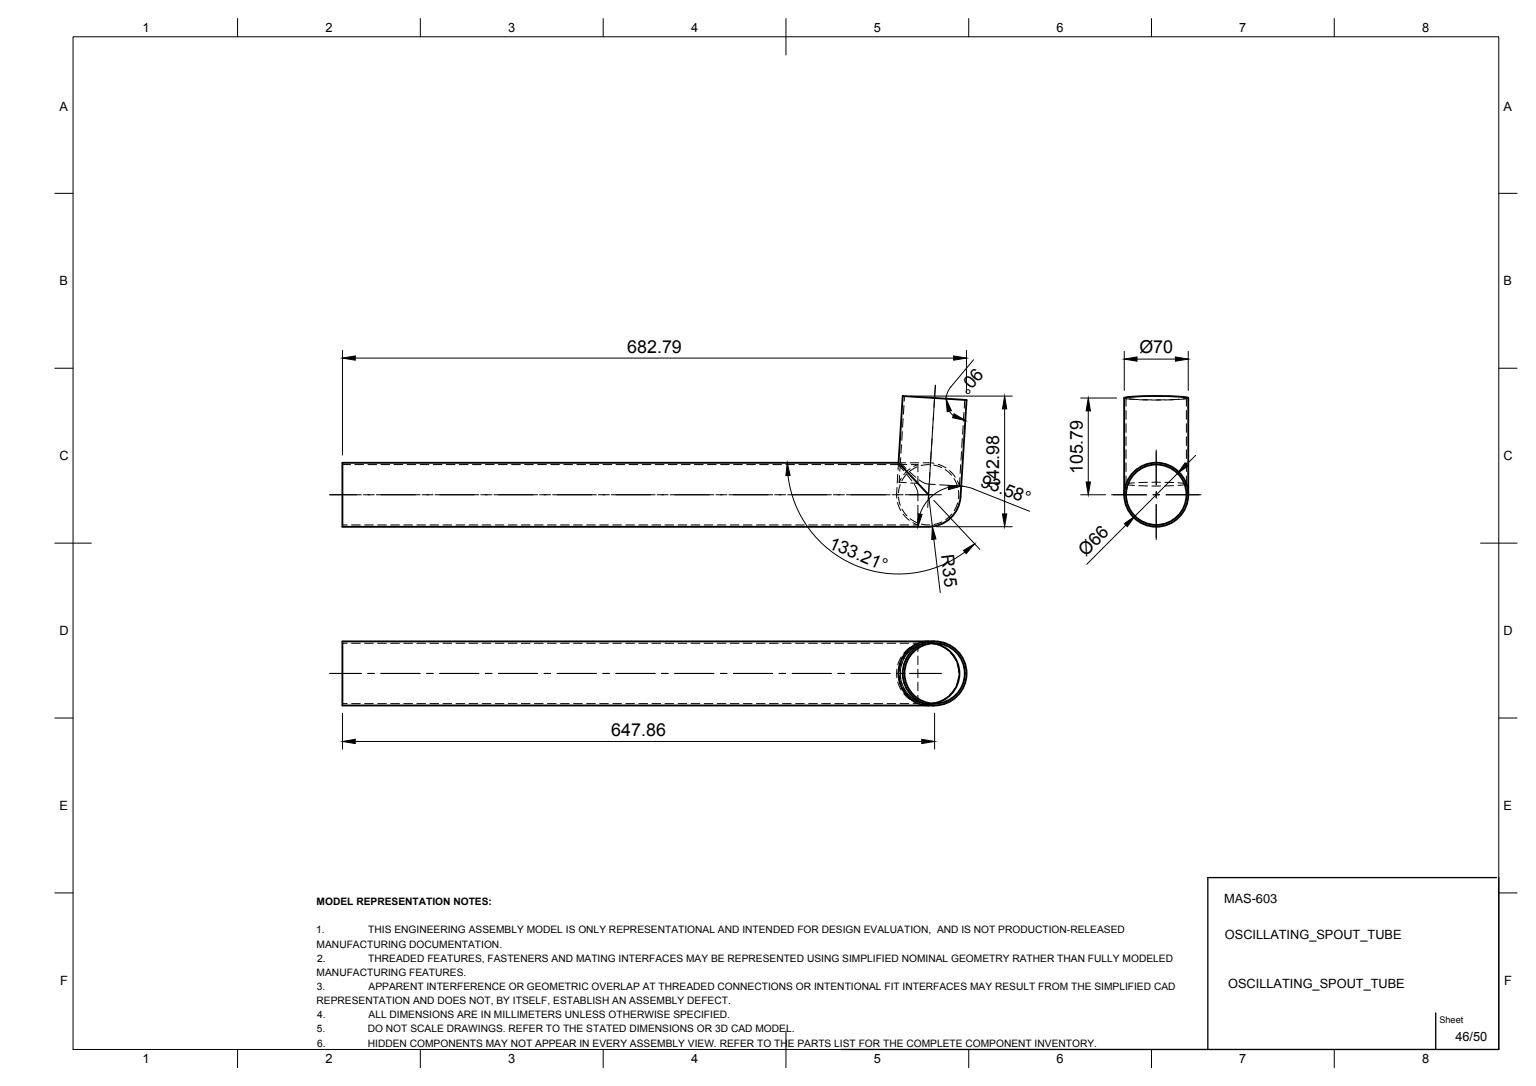
ISO-10303-21;
HEADER;
FILE_DESCRIPTION((''),'2;1');
FILE_NAME('OSCILLATING_SPOUT_TUBE.step','2026-10-01T22:06:14-07:00',(''),(''),'','','');
FILE_SCHEMA (('AUTOMOTIVE_DESIGN { 1 0 10303 214 3 1 1 }'));
ENDSEC;
DATA;
#10=MECHANICAL_DESIGN_GEOMETRIC_PRESENTATION_REPRESENTATION('',(#1021),#50440);
#36=B_SPLINE_CURVE_WITH_KNOTS('',3,(#49390,#49391,#49392,#49393,#49394,
#49395,#49396,#49397,#49398,#49399,#49400,#49401,#49402,#49403,#49404,#49405,
#49406,#49407,#49408,#49409,#49410,#49411,#49412,#49413,#49414,#49415,#49416,
#49417,#49418,#49419,#49420,#49421,#49422,#49423,#49424,#49425,#49426,#49427),
 .UNSPECIFIED.,.F.,.F.,(4,2,2,2,2,2,2,2,2,2,2,2,2,2,2,2,2,2,4),(11.701609895415,
11.9954810277209,12.363235333761,13.0987439458412,13.8342525579214,14.5697611700016,
15.2442090288987,15.9186568877959,16.593104746693,17.2675526055902,17.9420004644874,
18.6164483233845,19.2908961822817,19.9653440411788,20.700852653259,21.4363612653392,
22.1718698774194,22.5396241834595,22.8334953157654),.UNSPECIFIED.) ;
#37=B_SPLINE_CURVE_WITH_KNOTS('',3,(#49445,#49446,#49447,#49448,#49449,
#49450,#49451,#49452,#49453,#49454,#49455,#49456,#49457,#49458,#49459,#49460,
#49461,#49462,#49463,#49464,#49465,#49466,#49467,#49468,#49469,#49470,#49471,
#49472,#49473,#49474,#49475,#49476,#49477,#49478,#49479,#49480,#49481,#49482),
 .UNSPECIFIED.,.F.,.F.,(4,2,2,2,2,2,2,2,2,2,2,2,2,2,2,2,2,2,4),(0.0738831737341421,
0.367754306040092,0.735508612080185,1.47101722416037,2.20652583624055,2.94203444832074,
3.61648230721789,4.29093016611505,4.9653780250122,5.63982588390936,6.31427374280651,
6.98872160170367,7.66316946060082,8.33761731949797,9.07312593157816,9.80863454365834,
10.5441431557385,10.9118974617786,11.2057685940846),.UNSPECIFIED.) ;
#77=ORIENTED_CLOSED_SHELL('',*,#28697,.F.) ;
#78=ORIENTED_CLOSED_SHELL('',*,#28698,.F.) ;
#81=BREP_WITH_VOIDS('OSCILLATING_SPOUT_TUBE',#28699,(#77,#78)) ;
#673=ELLIPSE('',#32089,4.52782199571862,3.3) ;
#674=ELLIPSE('',#32097,4.80223545000459,3.5) ;
#875=SPHERICAL_SURFACE('',#32083,3.3) ;
#876=SPHERICAL_SURFACE('',#32085,3.5) ;
#877=SPHERICAL_SURFACE('',#32114,3.5) ;
#878=SPHERICAL_SURFACE('',#32115,3.5) ;
#879=SPHERICAL_SURFACE('',#32116,3.5) ;
#924=SHAPE_REPRESENTATION_RELATIONSHIP('SRR','None',#50658,#969) ;
#969=ADVANCED_BREP_SHAPE_REPRESENTATION('',(#81),#50427) ;
#1021=STYLED_ITEM('',(#50889),#81) ;
#1388=FACE_BOUND('',#5587,.T.) ;
#1389=FACE_BOUND('',#5591,.T.) ;
#2256=PLANE('',#32091) ;
#2257=PLANE('',#32100) ;
#3752=FACE_OUTER_BOUND('',#5582,.T.) ;
#3753=FACE_OUTER_BOUND('',#5583,.T.) ;
#3754=FACE_OUTER_BOUND('',#5584,.T.) ;
#3755=FACE_OUTER_BOUND('',#5585,.T.) ;
#3756=FACE_OUTER_BOUND('',#5586,.T.) ;
#3757=FACE_OUTER_BOUND('',#5588,.T.) ;
#3758=FACE_OUTER_BOUND('',#5589,.T.) ;
#3759=FACE_OUTER_BOUND('',#5590,.T.) ;
#3760=FACE_OUTER_BOUND('',#5592,.T.) ;
#3761=FACE_OUTER_BOUND('',#5593,.T.) ;
#3762=FACE_OUTER_BOUND('',#5594,.T.) ;
#3763=FACE_OUTER_BOUND('',#5595,.T.) ;
#3764=FACE_OUTER_BOUND('',#5596,.T.) ;
#3765=FACE_OUTER_BOUND('',#5597,.T.) ;
#3766=FACE_OUTER_BOUND('',#5598,.T.) ;
#5582=EDGE_LOOP('',(#26027,#26028)) ;
#5583=EDGE_LOOP('',(#26029,#26030)) ;
#5584=EDGE_LOOP('',(#26031,#26032)) ;
#5585=EDGE_LOOP('',(#26033,#26034)) ;
#5586=EDGE_LOOP('',(#26035)) ;
#5587=EDGE_LOOP('',(#26036)) ;
#5588=EDGE_LOOP('',(#26037,#26038)) ;
#5589=EDGE_LOOP('',(#26039,#26040,#26041,#26042,#26043,#26044)) ;
#5590=EDGE_LOOP('',(#26045)) ;
#5591=EDGE_LOOP('',(#26046)) ;
#5592=EDGE_LOOP('',(#26047,#26048)) ;
#5593=EDGE_LOOP('',(#26049,#26050,#26051,#26052,#26053,#26054)) ;
#5594=EDGE_LOOP('',(#26055,#26056,#26057,#26058,#26059,#26060)) ;
#5595=EDGE_LOOP('',(#26061,#26062,#26063,#26064,#26065,#26066)) ;
#5596=EDGE_LOOP('',(#26067,#26068,#26069)) ;
#5597=EDGE_LOOP('',(#26070,#26071,#26072,#26073)) ;
#5598=EDGE_LOOP('',(#26074,#26075,#26076,#26077,#26078)) ;
#8039=LINE('',#49435,#10511) ;
#8040=LINE('',#49486,#10512) ;
#8041=LINE('',#49492,#10513) ;
#8042=LINE('',#49496,#10514) ;
#10511=VECTOR('',#40462,3.5) ;
#10512=VECTOR('',#40477,3.5) ;
#10513=VECTOR('',#40486,3.3) ;
#10514=VECTOR('',#40491,3.3) ;
#11759=CIRCLE('',#32084,3.3) ;
#11760=CIRCLE('',#32086,3.3) ;
#11761=CIRCLE('',#32087,3.3) ;
#11762=CIRCLE('',#32092,3.5) ;
#11763=CIRCLE('',#32093,3.3) ;
#11764=CIRCLE('',#32095,3.5) ;
#11765=CIRCLE('',#32098,3.5) ;
#11766=CIRCLE('',#32099,3.5) ;
#11767=CIRCLE('',#32101,3.5) ;
#11768=CIRCLE('',#32102,3.3) ;
#11769=CIRCLE('',#32104,3.5) ;
#11770=CIRCLE('',#32106,3.5) ;
#11771=CIRCLE('',#32107,3.5) ;
#11772=CIRCLE('',#32109,3.3) ;
#11773=CIRCLE('',#32110,3.3) ;
#11774=CIRCLE('',#32112,3.3) ;
#11775=CIRCLE('',#32113,3.3) ;
#11776=CIRCLE('',#32117,3.5) ;
#14351=VERTEX_POINT('',#49371) ;
#14352=VERTEX_POINT('',#49372) ;
#14353=VERTEX_POINT('',#49375) ;
#14354=VERTEX_POINT('',#49376) ;
#14355=VERTEX_POINT('',#49383) ;
#14356=VERTEX_POINT('',#49385) ;
#14357=VERTEX_POINT('',#49388) ;
#14358=VERTEX_POINT('',#49389) ;
#14359=VERTEX_POINT('',#49430) ;
#14360=VERTEX_POINT('',#49431) ;
#14361=VERTEX_POINT('',#49433) ;
#14362=VERTEX_POINT('',#49438) ;
#14363=VERTEX_POINT('',#49440) ;
#14364=VERTEX_POINT('',#49443) ;
#14365=VERTEX_POINT('',#49444) ;
#14366=VERTEX_POINT('',#49485) ;
#14367=VERTEX_POINT('',#49490) ;
#14368=VERTEX_POINT('',#49495) ;
#14369=VERTEX_POINT('',#49502) ;
#18279=EDGE_CURVE('',#14351,#14352,#11759,.T.) ;
#18280=EDGE_CURVE('',#14353,#14354,#11760,.T.) ;
#18281=EDGE_CURVE('',#14354,#14353,#11761,.T.) ;
#18282=EDGE_CURVE('',#14353,#14354,#673,.T.) ;
#18283=EDGE_CURVE('',#14355,#14355,#11762,.T.) ;
#18284=EDGE_CURVE('',#14356,#14356,#11763,.T.) ;
#18285=EDGE_CURVE('',#14357,#14358,#36,.T.) ;
#18286=EDGE_CURVE('',#14357,#14358,#11764,.T.) ;
#18287=EDGE_CURVE('',#14359,#14360,#674,.T.) ;
#18288=EDGE_CURVE('',#14361,#14360,#11765,.T.) ;
#18289=EDGE_CURVE('',#14361,#14355,#8039,.T.) ;
#18290=EDGE_CURVE('',#14359,#14361,#11766,.T.) ;
#18291=EDGE_CURVE('',#14362,#14362,#11767,.T.) ;
#18292=EDGE_CURVE('',#14363,#14363,#11768,.T.) ;
#18293=EDGE_CURVE('',#14364,#14365,#37,.T.) ;
#18294=EDGE_CURVE('',#14365,#14364,#11769,.T.) ;
#18295=EDGE_CURVE('',#14362,#14366,#8040,.T.) ;
#18296=EDGE_CURVE('',#14360,#14366,#11770,.T.) ;
#18297=EDGE_CURVE('',#14366,#14359,#11771,.T.) ;
#18298=EDGE_CURVE('',#14357,#14367,#11772,.T.) ;
#18299=EDGE_CURVE('',#14367,#14363,#8041,.T.) ;
#18300=EDGE_CURVE('',#14367,#14358,#11773,.T.) ;
#18301=EDGE_CURVE('',#14356,#14368,#8042,.T.) ;
#18302=EDGE_CURVE('',#14368,#14364,#11774,.T.) ;
#18303=EDGE_CURVE('',#14365,#14368,#11775,.T.) ;
#18304=EDGE_CURVE('',#14369,#14368,#11776,.T.) ;
#26027=ORIENTED_EDGE('',*,*,#18279,.T.) ;
#26028=ORIENTED_EDGE('',*,*,#18279,.F.) ;
#26029=ORIENTED_EDGE('',*,*,#18280,.F.) ;
#26030=ORIENTED_EDGE('',*,*,#18281,.F.) ;
#26031=ORIENTED_EDGE('',*,*,#18281,.T.) ;
#26032=ORIENTED_EDGE('',*,*,#18282,.T.) ;
#26033=ORIENTED_EDGE('',*,*,#18280,.T.) ;
#26034=ORIENTED_EDGE('',*,*,#18282,.F.) ;
#26035=ORIENTED_EDGE('',*,*,#18283,.T.) ;
#26036=ORIENTED_EDGE('',*,*,#18284,.T.) ;
#26037=ORIENTED_EDGE('',*,*,#18285,.T.) ;
#26038=ORIENTED_EDGE('',*,*,#18286,.F.) ;
#26039=ORIENTED_EDGE('',*,*,#18287,.T.) ;
#26040=ORIENTED_EDGE('',*,*,#18288,.F.) ;
#26041=ORIENTED_EDGE('',*,*,#18289,.T.) ;
#26042=ORIENTED_EDGE('',*,*,#18283,.F.) ;
#26043=ORIENTED_EDGE('',*,*,#18289,.F.) ;
#26044=ORIENTED_EDGE('',*,*,#18290,.F.) ;
#26045=ORIENTED_EDGE('',*,*,#18291,.T.) ;
#26046=ORIENTED_EDGE('',*,*,#18292,.T.) ;
#26047=ORIENTED_EDGE('',*,*,#18293,.F.) ;
#26048=ORIENTED_EDGE('',*,*,#18294,.F.) ;
#26049=ORIENTED_EDGE('',*,*,#18291,.F.) ;
#26050=ORIENTED_EDGE('',*,*,#18295,.T.) ;
#26051=ORIENTED_EDGE('',*,*,#18296,.F.) ;
#26052=ORIENTED_EDGE('',*,*,#18287,.F.) ;
#26053=ORIENTED_EDGE('',*,*,#18297,.F.) ;
#26054=ORIENTED_EDGE('',*,*,#18295,.F.) ;
#26055=ORIENTED_EDGE('',*,*,#18298,.T.) ;
#26056=ORIENTED_EDGE('',*,*,#18299,.T.) ;
#26057=ORIENTED_EDGE('',*,*,#18292,.F.) ;
#26058=ORIENTED_EDGE('',*,*,#18299,.F.) ;
#26059=ORIENTED_EDGE('',*,*,#18300,.T.) ;
#26060=ORIENTED_EDGE('',*,*,#18285,.F.) ;
#26061=ORIENTED_EDGE('',*,*,#18284,.F.) ;
#26062=ORIENTED_EDGE('',*,*,#18301,.T.) ;
#26063=ORIENTED_EDGE('',*,*,#18302,.T.) ;
#26064=ORIENTED_EDGE('',*,*,#18293,.T.) ;
#26065=ORIENTED_EDGE('',*,*,#18303,.T.) ;
#26066=ORIENTED_EDGE('',*,*,#18301,.F.) ;
#26067=ORIENTED_EDGE('',*,*,#18298,.F.) ;
#26068=ORIENTED_EDGE('',*,*,#18286,.T.) ;
#26069=ORIENTED_EDGE('',*,*,#18300,.F.) ;
#26070=ORIENTED_EDGE('',*,*,#18296,.T.) ;
#26071=ORIENTED_EDGE('',*,*,#18297,.T.) ;
#26072=ORIENTED_EDGE('',*,*,#18290,.T.) ;
#26073=ORIENTED_EDGE('',*,*,#18288,.T.) ;
#26074=ORIENTED_EDGE('',*,*,#18294,.T.) ;
#26075=ORIENTED_EDGE('',*,*,#18302,.F.) ;
#26076=ORIENTED_EDGE('',*,*,#18304,.F.) ;
#26077=ORIENTED_EDGE('',*,*,#18304,.T.) ;
#26078=ORIENTED_EDGE('',*,*,#18303,.F.) ;
#27033=CYLINDRICAL_SURFACE('',#32088,3.3) ;
#27034=CYLINDRICAL_SURFACE('',#32090,3.3) ;
#27035=CYLINDRICAL_SURFACE('',#32094,3.5) ;
#27036=CYLINDRICAL_SURFACE('',#32096,3.5) ;
#27037=CYLINDRICAL_SURFACE('',#32103,3.5) ;
#27038=CYLINDRICAL_SURFACE('',#32105,3.5) ;
#27039=CYLINDRICAL_SURFACE('',#32108,3.3) ;
#27040=CYLINDRICAL_SURFACE('',#32111,3.3) ;
#28487=ADVANCED_FACE('',(#3752),#875,.F.) ;
#28488=ADVANCED_FACE('',(#3753),#876,.T.) ;
#28489=ADVANCED_FACE('',(#3754),#27033,.F.) ;
#28490=ADVANCED_FACE('',(#3755),#27034,.F.) ;
#28491=ADVANCED_FACE('',(#3756,#1388),#2256,.T.) ;
#28492=ADVANCED_FACE('',(#3757),#27035,.T.) ;
#28493=ADVANCED_FACE('',(#3758),#27036,.T.) ;
#28494=ADVANCED_FACE('',(#3759,#1389),#2257,.T.) ;
#28495=ADVANCED_FACE('',(#3760),#27037,.T.) ;
#28496=ADVANCED_FACE('',(#3761),#27038,.T.) ;
#28497=ADVANCED_FACE('',(#3762),#27039,.F.) ;
#28498=ADVANCED_FACE('',(#3763),#27040,.F.) ;
#28499=ADVANCED_FACE('',(#3764),#877,.T.) ;
#28500=ADVANCED_FACE('',(#3765),#878,.T.) ;
#28501=ADVANCED_FACE('',(#3766),#879,.T.) ;
#28697=CLOSED_SHELL('',(#28487)) ;
#28698=CLOSED_SHELL('',(#28488,#28489,#28490)) ;
#28699=CLOSED_SHELL('',(#28491,#28492,#28493,#28494,#28495,#28496,#28497,
#28498,#28499,#28500,#28501)) ;
#32082=AXIS2_PLACEMENT_3D('',#49369,#40428,#40429) ;
#32083=AXIS2_PLACEMENT_3D('',#49370,#40430,#40431) ;
#32084=AXIS2_PLACEMENT_3D('',#49373,#40432,#40433) ;
#32085=AXIS2_PLACEMENT_3D('',#49374,#40434,#40435) ;
#32086=AXIS2_PLACEMENT_3D('',#49377,#40436,#40437) ;
#32087=AXIS2_PLACEMENT_3D('',#49378,#40438,#40439) ;
#32088=AXIS2_PLACEMENT_3D('',#49379,#40440,#40441) ;
#32089=AXIS2_PLACEMENT_3D('',#49380,#40442,#40443) ;
#32090=AXIS2_PLACEMENT_3D('',#49381,#40444,#40445) ;
#32091=AXIS2_PLACEMENT_3D('',#49382,#40446,#40447) ;
#32092=AXIS2_PLACEMENT_3D('',#49384,#40448,#40449) ;
#32093=AXIS2_PLACEMENT_3D('',#49386,#40450,#40451) ;
#32094=AXIS2_PLACEMENT_3D('',#49387,#40452,#40453) ;
#32095=AXIS2_PLACEMENT_3D('',#49428,#40454,#40455) ;
#32096=AXIS2_PLACEMENT_3D('',#49429,#40456,#40457) ;
#32097=AXIS2_PLACEMENT_3D('',#49432,#40458,#40459) ;
#32098=AXIS2_PLACEMENT_3D('',#49434,#40460,#40461) ;
#32099=AXIS2_PLACEMENT_3D('',#49436,#40463,#40464) ;
#32100=AXIS2_PLACEMENT_3D('',#49437,#40465,#40466) ;
#32101=AXIS2_PLACEMENT_3D('',#49439,#40467,#40468) ;
#32102=AXIS2_PLACEMENT_3D('',#49441,#40469,#40470) ;
#32103=AXIS2_PLACEMENT_3D('',#49442,#40471,#40472) ;
#32104=AXIS2_PLACEMENT_3D('',#49483,#40473,#40474) ;
#32105=AXIS2_PLACEMENT_3D('',#49484,#40475,#40476) ;
#32106=AXIS2_PLACEMENT_3D('',#49487,#40478,#40479) ;
#32107=AXIS2_PLACEMENT_3D('',#49488,#40480,#40481) ;
#32108=AXIS2_PLACEMENT_3D('',#49489,#40482,#40483) ;
#32109=AXIS2_PLACEMENT_3D('',#49491,#40484,#40485) ;
#32110=AXIS2_PLACEMENT_3D('',#49493,#40487,#40488) ;
#32111=AXIS2_PLACEMENT_3D('',#49494,#40489,#40490) ;
#32112=AXIS2_PLACEMENT_3D('',#49497,#40492,#40493) ;
#32113=AXIS2_PLACEMENT_3D('',#49498,#40494,#40495) ;
#32114=AXIS2_PLACEMENT_3D('',#49499,#40496,#40497) ;
#32115=AXIS2_PLACEMENT_3D('',#49500,#40498,#40499) ;
#32116=AXIS2_PLACEMENT_3D('',#49501,#40500,#40501) ;
#32117=AXIS2_PLACEMENT_3D('',#49503,#40502,#40503) ;
#40428=DIRECTION('axis',(0.,0.,1.)) ;
#40429=DIRECTION('refdir',(1.,0.,0.)) ;
#40430=DIRECTION('center_axis',(6.12323399573676E-17,0.,1.)) ;
#40431=DIRECTION('ref_axis',(1.,0.,0.)) ;
#40432=DIRECTION('center_axis',(-1.22464679914735E-16,1.,0.)) ;
#40433=DIRECTION('ref_axis',(-1.,-1.22464679914735E-16,0.)) ;
#40434=DIRECTION('center_axis',(6.12323399573677E-17,0.,1.)) ;
#40435=DIRECTION('ref_axis',(1.,0.,0.)) ;
#40436=DIRECTION('center_axis',(-0.998052578482889,0.,0.0623782861551806)) ;
#40437=DIRECTION('ref_axis',(0.0623782861551814,0.,0.998052578482889)) ;
#40438=DIRECTION('center_axis',(0.,0.,-1.)) ;
#40439=DIRECTION('ref_axis',(1.,0.,0.)) ;
#40440=DIRECTION('center_axis',(0.,0.,-1.)) ;
#40441=DIRECTION('ref_axis',(1.,0.,0.)) ;
#40442=DIRECTION('center_axis',(-0.68469763905129,0.,0.728827238155648)) ;
#40443=DIRECTION('ref_axis',(0.728827238155648,0.,0.68469763905129)) ;
#40444=DIRECTION('center_axis',(0.998052578482889,0.,-0.0623782861551806)) ;
#40445=DIRECTION('ref_axis',(0.0623782861551806,0.,0.998052578482889)) ;
#40446=DIRECTION('center_axis',(0.,0.,1.)) ;
#40447=DIRECTION('ref_axis',(-1.,0.,0.)) ;
#40448=DIRECTION('center_axis',(0.,0.,1.)) ;
#40449=DIRECTION('ref_axis',(1.,0.,0.)) ;
#40450=DIRECTION('center_axis',(0.,0.,-1.)) ;
#40451=DIRECTION('ref_axis',(1.,0.,0.)) ;
#40452=DIRECTION('center_axis',(0.,0.,-1.)) ;
#40453=DIRECTION('ref_axis',(1.,0.,0.)) ;
#40454=DIRECTION('center_axis',(0.,0.,-1.)) ;
#40455=DIRECTION('ref_axis',(1.,0.,0.)) ;
#40456=DIRECTION('center_axis',(0.,0.,-1.)) ;
#40457=DIRECTION('ref_axis',(1.,0.,0.)) ;
#40458=DIRECTION('center_axis',(-0.68469763905129,0.,0.728827238155648)) ;
#40459=DIRECTION('ref_axis',(0.728827238155648,0.,0.68469763905129)) ;
#40460=DIRECTION('center_axis',(0.,0.,-1.)) ;
#40461=DIRECTION('ref_axis',(1.,0.,0.)) ;
#40462=DIRECTION('',(0.,0.,1.)) ;
#40463=DIRECTION('center_axis',(0.,0.,-1.)) ;
#40464=DIRECTION('ref_axis',(1.,0.,0.)) ;
#40465=DIRECTION('center_axis',(0.998052578482889,0.,-0.0623782861551805)) ;
#40466=DIRECTION('ref_axis',(0.0623782861551805,0.,0.998052578482889)) ;
#40467=DIRECTION('center_axis',(0.998052578482889,0.,-0.0623782861551805)) ;
#40468=DIRECTION('ref_axis',(0.0623782861551805,0.,0.998052578482889)) ;
#40469=DIRECTION('center_axis',(-0.998052578482889,0.,0.0623782861551805)) ;
#40470=DIRECTION('ref_axis',(0.0623782861551806,0.,0.998052578482889)) ;
#40471=DIRECTION('center_axis',(0.998052578482889,0.,-0.0623782861551805)) ;
#40472=DIRECTION('ref_axis',(0.0623782861551805,0.,0.998052578482889)) ;
#40473=DIRECTION('center_axis',(-0.998052578482889,0.,0.0623782861551805)) ;
#40474=DIRECTION('ref_axis',(0.0623782861551805,0.,0.998052578482889)) ;
#40475=DIRECTION('center_axis',(0.998052578482889,0.,-0.0623782861551805)) ;
#40476=DIRECTION('ref_axis',(0.0623782861551805,0.,0.998052578482889)) ;
#40477=DIRECTION('',(-0.998052578482889,0.,0.0623782861551805)) ;
#40478=DIRECTION('center_axis',(-0.998052578482889,0.,0.0623782861551805)) ;
#40479=DIRECTION('ref_axis',(0.0623782861551805,0.,0.998052578482889)) ;
#40480=DIRECTION('center_axis',(-0.998052578482889,0.,0.0623782861551805)) ;
#40481=DIRECTION('ref_axis',(0.0623782861551805,0.,0.998052578482889)) ;
#40482=DIRECTION('center_axis',(0.998052578482889,0.,-0.0623782861551806)) ;
#40483=DIRECTION('ref_axis',(0.0623782861551806,0.,0.998052578482889)) ;
#40484=DIRECTION('center_axis',(-0.998052578482889,0.,0.0623782861551806)) ;
#40485=DIRECTION('ref_axis',(0.0623782861551814,0.,0.998052578482889)) ;
#40486=DIRECTION('',(0.998052578482889,0.,-0.0623782861551806)) ;
#40487=DIRECTION('center_axis',(-0.998052578482889,0.,0.0623782861551806)) ;
#40488=DIRECTION('ref_axis',(0.0623782861551814,0.,0.998052578482889)) ;
#40489=DIRECTION('center_axis',(0.,0.,-1.)) ;
#40490=DIRECTION('ref_axis',(1.,0.,0.)) ;
#40491=DIRECTION('',(0.,0.,-1.)) ;
#40492=DIRECTION('center_axis',(0.,0.,-1.)) ;
#40493=DIRECTION('ref_axis',(1.,0.,0.)) ;
#40494=DIRECTION('center_axis',(0.,0.,-1.)) ;
#40495=DIRECTION('ref_axis',(1.,0.,0.)) ;
#40496=DIRECTION('center_axis',(6.12323399573677E-17,0.,1.)) ;
#40497=DIRECTION('ref_axis',(1.,0.,0.)) ;
#40498=DIRECTION('center_axis',(-6.12323399573677E-17,7.49879891330929E-33,
1.)) ;
#40499=DIRECTION('ref_axis',(-1.,1.22464679914735E-16,0.)) ;
#40500=DIRECTION('center_axis',(6.12323399573677E-17,0.,1.)) ;
#40501=DIRECTION('ref_axis',(1.,0.,0.)) ;
#40502=DIRECTION('center_axis',(1.22464679914735E-16,-1.,0.)) ;
#40503=DIRECTION('ref_axis',(-1.,-1.22464679914735E-16,0.)) ;
#49369=CARTESIAN_POINT('',(0.,0.,0.)) ;
#49370=CARTESIAN_POINT('Origin',(0.,0.,15.)) ;
#49371=CARTESIAN_POINT('',(-2.02066721859313E-16,-2.47460364139207E-32,
11.7)) ;
#49372=CARTESIAN_POINT('',(-2.02066721859313E-16,-2.47460364139207E-32,
18.3)) ;
#49373=CARTESIAN_POINT('Origin',(0.,0.,15.)) ;
#49374=CARTESIAN_POINT('Origin',(0.,0.,15.)) ;
#49375=CARTESIAN_POINT('',(1.24135277324074,-3.05762052785618,16.1661903789691)) ;
#49376=CARTESIAN_POINT('',(1.24135277324074,3.05762052785618,16.1661903789691)) ;
#49377=CARTESIAN_POINT('Origin',(1.16391931473201,0.,14.9272550428293)) ;
#49378=CARTESIAN_POINT('Origin',(0.,0.,16.1661903789691)) ;
#49379=CARTESIAN_POINT('Origin',(0.,0.,20.3)) ;
#49380=CARTESIAN_POINT('Origin',(-7.105427357601E-15,0.,15.)) ;
#49381=CARTESIAN_POINT('Origin',(32.,0.,13.)) ;
#49382=CARTESIAN_POINT('Origin',(0.,0.,25.6)) ;
#49383=CARTESIAN_POINT('',(-3.5,4.28626379701574E-16,25.6)) ;
#49384=CARTESIAN_POINT('Origin',(0.,0.,25.6)) ;
#49385=CARTESIAN_POINT('',(-3.3,4.04133443718627E-16,25.6)) ;
#49386=CARTESIAN_POINT('Origin',(0.,0.,25.6)) ;
#49387=CARTESIAN_POINT('Origin',(0.,0.,20.3)) ;
#49388=CARTESIAN_POINT('',(1.16846587455518,3.2991949775665,15.)) ;
#49389=CARTESIAN_POINT('',(1.16846587455518,-3.2991949775665,15.)) ;
#49390=CARTESIAN_POINT('Ctrl Pts',(1.16846587455518,3.2991949775665,15.)) ;
#49391=CARTESIAN_POINT('Ctrl Pts',(1.17442519254118,3.29708438399758,15.095349087776)) ;
#49392=CARTESIAN_POINT('Ctrl Pts',(1.19175023527009,3.29096616123353,15.1857170921028)) ;
#49393=CARTESIAN_POINT('Ctrl Pts',(1.24866258002262,3.26985933817832,15.3815376197941)) ;
#49394=CARTESIAN_POINT('Ctrl Pts',(1.29262895141202,3.25303416693559,15.4850971713711)) ;
#49395=CARTESIAN_POINT('Ctrl Pts',(1.44734056737426,3.18868022291068,15.7871365053987)) ;
#49396=CARTESIAN_POINT('Ctrl Pts',(1.57974867435124,3.12746840533713,15.9770140205015)) ;
#49397=CARTESIAN_POINT('Ctrl Pts',(1.86407692726612,2.96679654013783,16.3464498247156)) ;
#49398=CARTESIAN_POINT('Ctrl Pts',(2.01576973425023,2.86748054151594,16.5241537838072)) ;
#49399=CARTESIAN_POINT('Ctrl Pts',(2.3130389850849,2.63355709436769,16.8591337253863)) ;
#49400=CARTESIAN_POINT('Ctrl Pts',(2.45876907363751,2.49887177450341,17.0162189313947)) ;
#49401=CARTESIAN_POINT('Ctrl Pts',(2.71598418768332,2.2151714704621,17.2886907349084)) ;
#49402=CARTESIAN_POINT('Ctrl Pts',(2.83748562910909,2.05938117281354,17.4149058836929)) ;
#49403=CARTESIAN_POINT('Ctrl Pts',(3.05933295429687,1.71255872522277,17.6430565099933)) ;
#49404=CARTESIAN_POINT('Ctrl Pts',(3.15964506633327,1.52149772138736,17.744980961747)) ;
#49405=CARTESIAN_POINT('Ctrl Pts',(3.32517088360158,1.11424924967644,17.9123789095648)) ;
#49406=CARTESIAN_POINT('Ctrl Pts',(3.39053849186878,0.897553052697191,17.978012051174)) ;
#49407=CARTESIAN_POINT('Ctrl Pts',(3.47797144791113,0.452843632408543,18.0656854316297)) ;
#49408=CARTESIAN_POINT('Ctrl Pts',(3.5,0.224815952965719,18.087689030513)) ;
#49409=CARTESIAN_POINT('Ctrl Pts',(3.5,-0.224815952965717,18.087689030513)) ;
#49410=CARTESIAN_POINT('Ctrl Pts',(3.47797144791113,-0.452843632408542,
18.0656854316297)) ;
#49411=CARTESIAN_POINT('Ctrl Pts',(3.39053849186878,-0.89755305269719,17.978012051174)) ;
#49412=CARTESIAN_POINT('Ctrl Pts',(3.32517088360158,-1.11424924967644,17.9123789095648)) ;
#49413=CARTESIAN_POINT('Ctrl Pts',(3.15964506633327,-1.52149772138736,17.744980961747)) ;
#49414=CARTESIAN_POINT('Ctrl Pts',(3.05933295429687,-1.71255872522277,17.6430565099933)) ;
#49415=CARTESIAN_POINT('Ctrl Pts',(2.83748562910909,-2.05938117281353,17.4149058836929)) ;
#49416=CARTESIAN_POINT('Ctrl Pts',(2.71598418768332,-2.2151714704621,17.2886907349084)) ;
#49417=CARTESIAN_POINT('Ctrl Pts',(2.45876907363751,-2.49887177450341,17.0162189313947)) ;
#49418=CARTESIAN_POINT('Ctrl Pts',(2.31303898508491,-2.63355709436768,16.8591337253863)) ;
#49419=CARTESIAN_POINT('Ctrl Pts',(2.01576973425023,-2.86748054151594,16.5241537838072)) ;
#49420=CARTESIAN_POINT('Ctrl Pts',(1.86407692726612,-2.96679654013782,16.3464498247156)) ;
#49421=CARTESIAN_POINT('Ctrl Pts',(1.57974867435124,-3.12746840533713,15.9770140205015)) ;
#49422=CARTESIAN_POINT('Ctrl Pts',(1.44734056737426,-3.18868022291068,15.7871365053987)) ;
#49423=CARTESIAN_POINT('Ctrl Pts',(1.29262895141202,-3.25303416693559,15.4850971713711)) ;
#49424=CARTESIAN_POINT('Ctrl Pts',(1.24866258002262,-3.26985933817832,15.3815376197941)) ;
#49425=CARTESIAN_POINT('Ctrl Pts',(1.19175023527009,-3.29096616123353,15.1857170921028)) ;
#49426=CARTESIAN_POINT('Ctrl Pts',(1.17442519254118,-3.29708438399758,15.095349087776)) ;
#49427=CARTESIAN_POINT('Ctrl Pts',(1.16846587455518,-3.2991949775665,15.)) ;
#49428=CARTESIAN_POINT('Origin',(0.,0.,15.)) ;
#49429=CARTESIAN_POINT('Origin',(0.,0.,20.3)) ;
#49430=CARTESIAN_POINT('',(-7.13318293321663E-15,-3.5,15.)) ;
#49431=CARTESIAN_POINT('',(-7.13318293321663E-15,3.5,15.)) ;
#49432=CARTESIAN_POINT('Origin',(-7.105427357601E-15,0.,15.)) ;
#49433=CARTESIAN_POINT('',(-3.5,4.28626379701574E-16,15.)) ;
#49434=CARTESIAN_POINT('Origin',(0.,0.,15.)) ;
#49435=CARTESIAN_POINT('',(-3.5,4.28626379701574E-16,20.3)) ;
#49436=CARTESIAN_POINT('Origin',(0.,0.,15.)) ;
#49437=CARTESIAN_POINT('Origin',(64.,0.,11.)) ;
#49438=CARTESIAN_POINT('',(63.7816759984569,4.28626379701574E-16,7.50681597530989)) ;
#49439=CARTESIAN_POINT('Origin',(64.,0.,11.)) ;
#49440=CARTESIAN_POINT('',(63.7941516556879,-4.04133443718627E-16,7.70642649100647)) ;
#49441=CARTESIAN_POINT('Origin',(64.,0.,11.)) ;
#49442=CARTESIAN_POINT('Origin',(32.,0.,13.)) ;
#49443=CARTESIAN_POINT('',(0.0728868986855592,3.2991949775665,16.1661903789691)) ;
#49444=CARTESIAN_POINT('',(0.0728868986855592,-3.2991949775665,16.1661903789691)) ;
#49445=CARTESIAN_POINT('Ctrl Pts',(0.0728868986855593,3.2991949775665,16.1661903789691)) ;
#49446=CARTESIAN_POINT('Ctrl Pts',(0.168422033639041,3.29708438399758,16.1661903789691)) ;
#49447=CARTESIAN_POINT('Ctrl Pts',(0.259694759842746,3.29096616123353,16.1778446813038)) ;
#49448=CARTESIAN_POINT('Ctrl Pts',(0.458684036951621,3.26985933817832,16.2224312448202)) ;
#49449=CARTESIAN_POINT('Ctrl Pts',(0.564784461325359,3.25303416693559,16.2598521278095)) ;
#49450=CARTESIAN_POINT('Ctrl Pts',(0.87588624290687,3.18868022291068,16.3954217590338)) ;
#49451=CARTESIAN_POINT('Ctrl Pts',(1.07365337723744,3.12746840533713,16.5157277776427)) ;
#49452=CARTESIAN_POINT('Ctrl Pts',(1.46010564333952,2.96679654013783,16.7764575512887)) ;
#49453=CARTESIAN_POINT('Ctrl Pts',(1.64692587523926,2.86748054151594,16.9167700800254)) ;
#49454=CARTESIAN_POINT('Ctrl Pts',(1.99979661606603,2.63355709436769,17.1925649476725)) ;
#49455=CARTESIAN_POINT('Ctrl Pts',(2.16566630412932,2.49887177450341,17.3282125323839)) ;
#49456=CARTESIAN_POINT('Ctrl Pts',(2.45365212817748,2.2151714704621,17.5679304160533)) ;
#49457=CARTESIAN_POINT('Ctrl Pts',(2.58720053454703,2.05938117281353,17.6813221582896)) ;
#49458=CARTESIAN_POINT('Ctrl Pts',(2.82874531134193,1.71255872522277,17.888505808169)) ;
#49459=CARTESIAN_POINT('Ctrl Pts',(2.93672857085459,1.52149772138736,17.9822646976223)) ;
#49460=CARTESIAN_POINT('Ctrl Pts',(3.11412574110247,1.11424924967644,18.1370261692616)) ;
#49461=CARTESIAN_POINT('Ctrl Pts',(3.18370858669324,0.897553052697192,18.1981723963534)) ;
#49462=CARTESIAN_POINT('Ctrl Pts',(3.27666514807284,0.452843632408543,18.2799661683616)) ;
#49463=CARTESIAN_POINT('Ctrl Pts',(3.3,0.224815952965718,18.3005792747866)) ;
#49464=CARTESIAN_POINT('Ctrl Pts',(3.3,-0.224815952965718,18.3005792747866)) ;
#49465=CARTESIAN_POINT('Ctrl Pts',(3.27666514807284,-0.452843632408543,
18.2799661683616)) ;
#49466=CARTESIAN_POINT('Ctrl Pts',(3.18370858669324,-0.897553052697191,
18.1981723963534)) ;
#49467=CARTESIAN_POINT('Ctrl Pts',(3.11412574110247,-1.11424924967644,18.1370261692616)) ;
#49468=CARTESIAN_POINT('Ctrl Pts',(2.93672857085459,-1.52149772138736,17.9822646976223)) ;
#49469=CARTESIAN_POINT('Ctrl Pts',(2.82874531134193,-1.71255872522277,17.888505808169)) ;
#49470=CARTESIAN_POINT('Ctrl Pts',(2.58720053454702,-2.05938117281353,17.6813221582896)) ;
#49471=CARTESIAN_POINT('Ctrl Pts',(2.45365212817748,-2.2151714704621,17.5679304160533)) ;
#49472=CARTESIAN_POINT('Ctrl Pts',(2.16566630412932,-2.49887177450341,17.3282125323839)) ;
#49473=CARTESIAN_POINT('Ctrl Pts',(1.99979661606603,-2.63355709436769,17.1925649476725)) ;
#49474=CARTESIAN_POINT('Ctrl Pts',(1.64692587523926,-2.86748054151594,16.9167700800254)) ;
#49475=CARTESIAN_POINT('Ctrl Pts',(1.46010564333952,-2.96679654013783,16.7764575512887)) ;
#49476=CARTESIAN_POINT('Ctrl Pts',(1.07365337723744,-3.12746840533713,16.5157277776427)) ;
#49477=CARTESIAN_POINT('Ctrl Pts',(0.87588624290687,-3.18868022291068,16.3954217590338)) ;
#49478=CARTESIAN_POINT('Ctrl Pts',(0.564784461325359,-3.25303416693559,
16.2598521278095)) ;
#49479=CARTESIAN_POINT('Ctrl Pts',(0.458684036951621,-3.26985933817832,
16.2224312448202)) ;
#49480=CARTESIAN_POINT('Ctrl Pts',(0.259694759842746,-3.29096616123353,
16.1778446813038)) ;
#49481=CARTESIAN_POINT('Ctrl Pts',(0.168422033639041,-3.29708438399758,
16.1661903789691)) ;
#49482=CARTESIAN_POINT('Ctrl Pts',(0.0728868986855591,-3.2991949775665,
16.1661903789691)) ;
#49483=CARTESIAN_POINT('Origin',(-7.105427357601E-15,0.,15.)) ;
#49484=CARTESIAN_POINT('Origin',(32.,0.,13.)) ;
#49485=CARTESIAN_POINT('',(-0.218324001543145,4.28626379701574E-16,11.5068159753099)) ;
#49486=CARTESIAN_POINT('',(31.7816759984569,4.28626379701574E-16,9.50681597530989)) ;
#49487=CARTESIAN_POINT('Origin',(-7.105427357601E-15,0.,15.)) ;
#49488=CARTESIAN_POINT('Origin',(-7.105427357601E-15,0.,15.)) ;
#49489=CARTESIAN_POINT('Origin',(32.,0.,13.)) ;
#49490=CARTESIAN_POINT('',(0.9580709704199,4.04133443718627E-16,11.6336815338357)) ;
#49491=CARTESIAN_POINT('Origin',(1.16391931473201,0.,14.9272550428293)) ;
#49492=CARTESIAN_POINT('',(31.7941516556879,4.04133443718627E-16,9.70642649100647)) ;
#49493=CARTESIAN_POINT('Origin',(1.16391931473201,0.,14.9272550428293)) ;
#49494=CARTESIAN_POINT('Origin',(0.,0.,20.3)) ;
#49495=CARTESIAN_POINT('',(-3.3,4.04133443718627E-16,16.1661903789691)) ;
#49496=CARTESIAN_POINT('',(-3.3,4.04133443718627E-16,20.3)) ;
#49497=CARTESIAN_POINT('Origin',(0.,0.,16.1661903789691)) ;
#49498=CARTESIAN_POINT('Origin',(0.,0.,16.1661903789691)) ;
#49499=CARTESIAN_POINT('Origin',(0.,0.,15.)) ;
#49500=CARTESIAN_POINT('Origin',(0.,0.,15.)) ;
#49501=CARTESIAN_POINT('Origin',(0.,0.,15.)) ;
#49502=CARTESIAN_POINT('',(-2.14313189850787E-16,-2.62457961965825E-32,
18.5)) ;
#49503=CARTESIAN_POINT('Origin',(0.,0.,15.)) ;
#50374=UNCERTAINTY_MEASURE_WITH_UNIT(LENGTH_MEASURE(0.001),#50441,
'DISTANCE_ACCURACY_VALUE',
'Maximum model space distance between geometric entities at asserted c
onnectivities') ;
#50387=UNCERTAINTY_MEASURE_WITH_UNIT(LENGTH_MEASURE(0.001),#50441,
'DISTANCE_ACCURACY_VALUE',
'Maximum model space distance between geometric entities at asserted c
onnectivities') ;
#50427=(
GEOMETRIC_REPRESENTATION_CONTEXT(3)
GLOBAL_UNCERTAINTY_ASSIGNED_CONTEXT((#50374))
GLOBAL_UNIT_ASSIGNED_CONTEXT((#50441,#50443,#50444))
REPRESENTATION_CONTEXT('','3D')
) ;
#50440=(
GEOMETRIC_REPRESENTATION_CONTEXT(3)
GLOBAL_UNCERTAINTY_ASSIGNED_CONTEXT((#50387))
GLOBAL_UNIT_ASSIGNED_CONTEXT((#50441,#50443,#50444))
REPRESENTATION_CONTEXT('','3D')
) ;
#50441=(
LENGTH_UNIT()
NAMED_UNIT(*)
SI_UNIT(.CENTI.,.METRE.)
) ;
#50443=(
NAMED_UNIT(*)
PLANE_ANGLE_UNIT()
SI_UNIT($,.RADIAN.)
) ;
#50444=(
NAMED_UNIT(*)
SI_UNIT($,.STERADIAN.)
SOLID_ANGLE_UNIT()
) ;
#50484=SHAPE_DEFINITION_REPRESENTATION(#50574,#50658) ;
#50574=PRODUCT_DEFINITION_SHAPE('',$,#50711) ;
#50658=SHAPE_REPRESENTATION('',(#32082),#50427) ;
#50671=PRODUCT_DEFINITION_CONTEXT('part definition',#50829,'design') ;
#50711=PRODUCT_DEFINITION('OSCILLATING_SPOUT_TUBE',
'OSCILLATING_SPOUT_TUBE',#50763,#50671) ;
#50763=PRODUCT_DEFINITION_FORMATION('',$,#50870) ;
#50829=APPLICATION_CONTEXT(
'Core Data for Automotive Mechanical Design Process') ;
#50830=PRODUCT_CONTEXT('part definition',#50829,'mechanical') ;
#50870=PRODUCT('OSCILLATING_SPOUT_TUBE','OSCILLATING_SPOUT_TUBE',$,(#50830)) ;
#50889=PRESENTATION_STYLE_ASSIGNMENT((#50896)) ;
#50896=SURFACE_STYLE_USAGE(.BOTH.,#50903) ;
#50903=SURFACE_SIDE_STYLE('',(#50910)) ;
#50910=SURFACE_STYLE_FILL_AREA(#50917) ;
#50917=FILL_AREA_STYLE('Stainless Steel - Satin',(#50924)) ;
#50924=FILL_AREA_STYLE_COLOUR('Stainless Steel - Satin',#50931) ;
#50931=COLOUR_RGB('Stainless Steel - Satin', 0.72549020, 0.75294118, 0.79215686) ;
ENDSEC;
END-ISO-10303-21;
